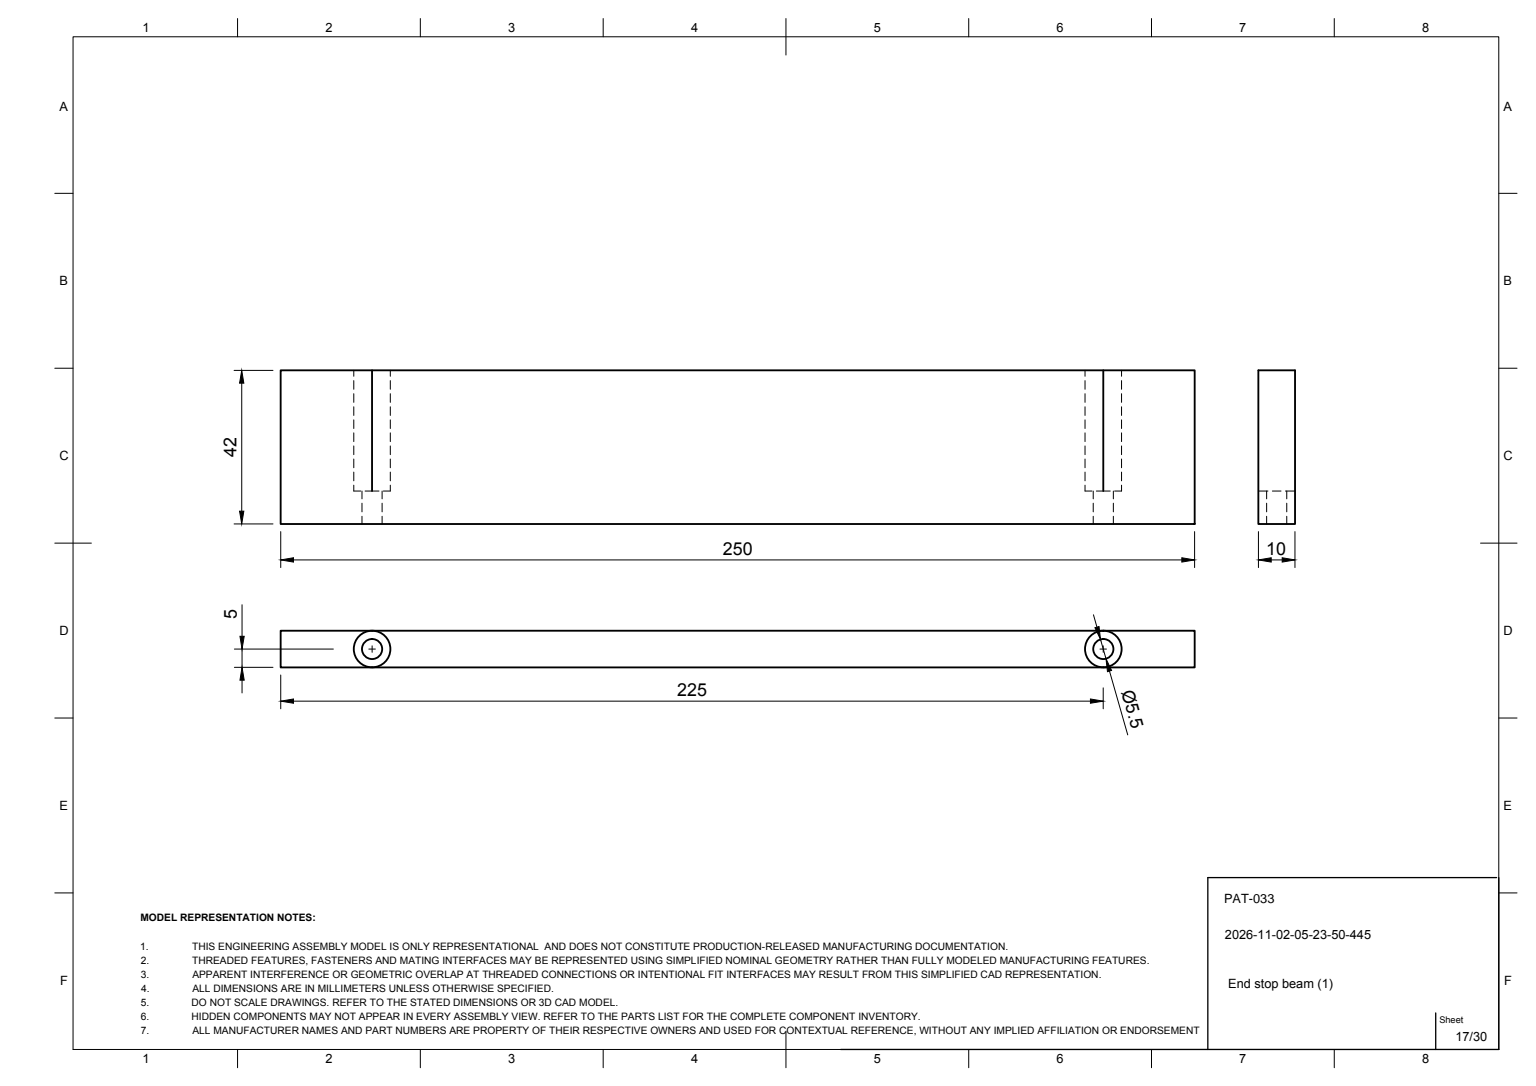
ISO-10303-21;
HEADER;
/* Generated by software containing ST-Developer
 * from STEP Tools, Inc. (www.steptools.com) 
 */

FILE_DESCRIPTION(
/* description */ ('Dual-rail gantry carriage'),
/* implementation_level */ '2;1');

FILE_NAME(
/* name */ 'End stop beam (1).step',
/* time_stamp */ '2026-10-27T10:49:15-07:00',
/* author */ (''),
/* organization */ (''),
/* preprocessor_version */ 'ST-DEVELOPER v20.2',
/* originating_system */ 'Autodesk Translation Framework v15.17.0.0',
/* authorisation */ '');

FILE_SCHEMA (('AUTOMOTIVE_DESIGN { 1 0 10303 214 3 1 1 }'));
ENDSEC;

DATA;
#10=MECHANICAL_DESIGN_GEOMETRIC_PRESENTATION_REPRESENTATION('',(#597),#12804);
#535=SHAPE_REPRESENTATION_RELATIONSHIP('SRR','None',#13013,#566);
#566=ADVANCED_BREP_SHAPE_REPRESENTATION('',(#628),#12783);
#597=STYLED_ITEM('',(#13233),#628);
#628=MANIFOLD_SOLID_BREP('Body1',#7375);
#686=FACE_BOUND('',#1586,.T.);
#687=FACE_BOUND('',#1590,.T.);
#688=FACE_BOUND('',#1601,.T.);
#689=FACE_BOUND('',#1602,.T.);
#840=PLANE('',#7916);
#841=PLANE('',#7924);
#842=PLANE('',#7926);
#843=PLANE('',#7927);
#844=PLANE('',#7928);
#845=PLANE('',#7933);
#846=PLANE('',#7934);
#847=PLANE('',#7935);
#848=PLANE('',#7936);
#849=PLANE('',#7937);
#1150=FACE_OUTER_BOUND('',#1583,.T.);
#1151=FACE_OUTER_BOUND('',#1584,.T.);
#1152=FACE_OUTER_BOUND('',#1585,.T.);
#1153=FACE_OUTER_BOUND('',#1587,.T.);
#1154=FACE_OUTER_BOUND('',#1588,.T.);
#1155=FACE_OUTER_BOUND('',#1589,.T.);
#1156=FACE_OUTER_BOUND('',#1591,.T.);
#1157=FACE_OUTER_BOUND('',#1592,.T.);
#1158=FACE_OUTER_BOUND('',#1593,.T.);
#1159=FACE_OUTER_BOUND('',#1594,.T.);
#1160=FACE_OUTER_BOUND('',#1595,.T.);
#1161=FACE_OUTER_BOUND('',#1596,.T.);
#1162=FACE_OUTER_BOUND('',#1597,.T.);
#1163=FACE_OUTER_BOUND('',#1598,.T.);
#1164=FACE_OUTER_BOUND('',#1599,.T.);
#1165=FACE_OUTER_BOUND('',#1600,.T.);
#1583=EDGE_LOOP('',(#5527,#5528,#5529,#5530));
#1584=EDGE_LOOP('',(#5531,#5532,#5533,#5534));
#1585=EDGE_LOOP('',(#5535,#5536));
#1586=EDGE_LOOP('',(#5537));
#1587=EDGE_LOOP('',(#5538,#5539,#5540,#5541));
#1588=EDGE_LOOP('',(#5542,#5543,#5544,#5545));
#1589=EDGE_LOOP('',(#5546,#5547));
#1590=EDGE_LOOP('',(#5548));
#1591=EDGE_LOOP('',(#5549,#5550,#5551,#5552));
#1592=EDGE_LOOP('',(#5553,#5554,#5555,#5556));
#1593=EDGE_LOOP('',(#5557,#5558,#5559,#5560));
#1594=EDGE_LOOP('',(#5561,#5562,#5563,#5564));
#1595=EDGE_LOOP('',(#5565,#5566,#5567,#5568));
#1596=EDGE_LOOP('',(#5569,#5570,#5571,#5572));
#1597=EDGE_LOOP('',(#5573,#5574,#5575,#5576,#5577,#5578,#5579,#5580,#5581,
#5582));
#1598=EDGE_LOOP('',(#5583,#5584,#5585,#5586));
#1599=EDGE_LOOP('',(#5587,#5588,#5589,#5590,#5591,#5592,#5593,#5594,#5595,
#5596));
#1600=EDGE_LOOP('',(#5597,#5598,#5599,#5600));
#1601=EDGE_LOOP('',(#5601));
#1602=EDGE_LOOP('',(#5602));
#2126=LINE('',#11186,#2835);
#2127=LINE('',#11190,#2836);
#2128=LINE('',#11193,#2837);
#2129=LINE('',#11195,#2838);
#2130=LINE('',#11203,#2839);
#2131=LINE('',#11207,#2840);
#2132=LINE('',#11210,#2841);
#2133=LINE('',#11212,#2842);
#2134=LINE('',#11219,#2843);
#2135=LINE('',#11221,#2844);
#2136=LINE('',#11222,#2845);
#2137=LINE('',#11224,#2846);
#2138=LINE('',#11225,#2847);
#2139=LINE('',#11228,#2848);
#2140=LINE('',#11230,#2849);
#2141=LINE('',#11231,#2850);
#2142=LINE('',#11235,#2851);
#2143=LINE('',#11239,#2852);
#2144=LINE('',#11243,#2853);
#2145=LINE('',#11244,#2854);
#2146=LINE('',#11245,#2855);
#2147=LINE('',#11248,#2856);
#2148=LINE('',#11249,#2857);
#2149=LINE('',#11252,#2858);
#2150=LINE('',#11253,#2859);
#2151=LINE('',#11255,#2860);
#2835=VECTOR('',#9005,1.);
#2836=VECTOR('',#9008,1.);
#2837=VECTOR('',#9013,1.);
#2838=VECTOR('',#9016,1.);
#2839=VECTOR('',#9025,1.);
#2840=VECTOR('',#9028,1.);
#2841=VECTOR('',#9033,1.);
#2842=VECTOR('',#9036,1.);
#2843=VECTOR('',#9045,1.);
#2844=VECTOR('',#9046,1.);
#2845=VECTOR('',#9047,1.);
#2846=VECTOR('',#9050,1.);
#2847=VECTOR('',#9051,1.);
#2848=VECTOR('',#9054,1.);
#2849=VECTOR('',#9055,1.);
#2850=VECTOR('',#9056,1.);
#2851=VECTOR('',#9061,0.274999999999999);
#2852=VECTOR('',#9066,0.274999999999999);
#2853=VECTOR('',#9069,1.);
#2854=VECTOR('',#9070,1.);
#2855=VECTOR('',#9071,1.);
#2856=VECTOR('',#9074,1.);
#2857=VECTOR('',#9075,1.);
#2858=VECTOR('',#9078,1.);
#2859=VECTOR('',#9079,1.);
#2860=VECTOR('',#9082,1.);
#3418=CIRCLE('',#7911,0.5);
#3419=CIRCLE('',#7912,0.5);
#3420=CIRCLE('',#7914,0.5);
#3421=CIRCLE('',#7915,0.5);
#3422=CIRCLE('',#7917,0.274999999999999);
#3423=CIRCLE('',#7919,0.5);
#3424=CIRCLE('',#7920,0.5);
#3425=CIRCLE('',#7922,0.5);
#3426=CIRCLE('',#7923,0.5);
#3427=CIRCLE('',#7925,0.274999999999999);
#3428=CIRCLE('',#7930,0.274999999999999);
#3429=CIRCLE('',#7932,0.274999999999999);
#3714=VERTEX_POINT('',#11184);
#3715=VERTEX_POINT('',#11185);
#3716=VERTEX_POINT('',#11187);
#3717=VERTEX_POINT('',#11189);
#3718=VERTEX_POINT('',#11198);
#3719=VERTEX_POINT('',#11201);
#3720=VERTEX_POINT('',#11202);
#3721=VERTEX_POINT('',#11204);
#3722=VERTEX_POINT('',#11206);
#3723=VERTEX_POINT('',#11215);
#3724=VERTEX_POINT('',#11218);
#3725=VERTEX_POINT('',#11220);
#3726=VERTEX_POINT('',#11227);
#3727=VERTEX_POINT('',#11229);
#3728=VERTEX_POINT('',#11233);
#3729=VERTEX_POINT('',#11237);
#3730=VERTEX_POINT('',#11241);
#3731=VERTEX_POINT('',#11242);
#3732=VERTEX_POINT('',#11247);
#3733=VERTEX_POINT('',#11251);
#4386=EDGE_CURVE('',#3714,#3715,#2126,.T.);
#4387=EDGE_CURVE('',#3716,#3715,#3418,.T.);
#4388=EDGE_CURVE('',#3717,#3716,#2127,.T.);
#4389=EDGE_CURVE('',#3714,#3717,#3419,.T.);
#4390=EDGE_CURVE('',#3714,#3715,#2128,.T.);
#4391=EDGE_CURVE('',#3717,#3714,#3420,.T.);
#4392=EDGE_CURVE('',#3717,#3716,#2129,.T.);
#4393=EDGE_CURVE('',#3715,#3716,#3421,.T.);
#4394=EDGE_CURVE('',#3718,#3718,#3422,.T.);
#4395=EDGE_CURVE('',#3719,#3720,#2130,.T.);
#4396=EDGE_CURVE('',#3721,#3720,#3423,.T.);
#4397=EDGE_CURVE('',#3722,#3721,#2131,.T.);
#4398=EDGE_CURVE('',#3719,#3722,#3424,.T.);
#4399=EDGE_CURVE('',#3719,#3720,#2132,.T.);
#4400=EDGE_CURVE('',#3722,#3719,#3425,.T.);
#4401=EDGE_CURVE('',#3722,#3721,#2133,.T.);
#4402=EDGE_CURVE('',#3720,#3721,#3426,.T.);
#4403=EDGE_CURVE('',#3723,#3723,#3427,.T.);
#4404=EDGE_CURVE('',#3720,#3724,#2134,.T.);
#4405=EDGE_CURVE('',#3724,#3725,#2135,.T.);
#4406=EDGE_CURVE('',#3725,#3721,#2136,.T.);
#4407=EDGE_CURVE('',#3715,#3720,#2137,.T.);
#4408=EDGE_CURVE('',#3721,#3716,#2138,.T.);
#4409=EDGE_CURVE('',#3716,#3726,#2139,.T.);
#4410=EDGE_CURVE('',#3726,#3727,#2140,.T.);
#4411=EDGE_CURVE('',#3727,#3715,#2141,.T.);
#4412=EDGE_CURVE('',#3728,#3728,#3428,.T.);
#4413=EDGE_CURVE('',#3728,#3718,#2142,.T.);
#4414=EDGE_CURVE('',#3729,#3729,#3429,.T.);
#4415=EDGE_CURVE('',#3729,#3723,#2143,.T.);
#4416=EDGE_CURVE('',#3730,#3731,#2144,.T.);
#4417=EDGE_CURVE('',#3731,#3725,#2145,.T.);
#4418=EDGE_CURVE('',#3730,#3724,#2146,.T.);
#4419=EDGE_CURVE('',#3732,#3730,#2147,.T.);
#4420=EDGE_CURVE('',#3732,#3727,#2148,.T.);
#4421=EDGE_CURVE('',#3733,#3732,#2149,.T.);
#4422=EDGE_CURVE('',#3733,#3726,#2150,.T.);
#4423=EDGE_CURVE('',#3731,#3733,#2151,.T.);
#5527=ORIENTED_EDGE('',*,*,#4386,.T.);
#5528=ORIENTED_EDGE('',*,*,#4387,.F.);
#5529=ORIENTED_EDGE('',*,*,#4388,.F.);
#5530=ORIENTED_EDGE('',*,*,#4389,.F.);
#5531=ORIENTED_EDGE('',*,*,#4390,.F.);
#5532=ORIENTED_EDGE('',*,*,#4391,.F.);
#5533=ORIENTED_EDGE('',*,*,#4392,.T.);
#5534=ORIENTED_EDGE('',*,*,#4393,.F.);
#5535=ORIENTED_EDGE('',*,*,#4391,.T.);
#5536=ORIENTED_EDGE('',*,*,#4389,.T.);
#5537=ORIENTED_EDGE('',*,*,#4394,.F.);
#5538=ORIENTED_EDGE('',*,*,#4395,.T.);
#5539=ORIENTED_EDGE('',*,*,#4396,.F.);
#5540=ORIENTED_EDGE('',*,*,#4397,.F.);
#5541=ORIENTED_EDGE('',*,*,#4398,.F.);
#5542=ORIENTED_EDGE('',*,*,#4399,.F.);
#5543=ORIENTED_EDGE('',*,*,#4400,.F.);
#5544=ORIENTED_EDGE('',*,*,#4401,.T.);
#5545=ORIENTED_EDGE('',*,*,#4402,.F.);
#5546=ORIENTED_EDGE('',*,*,#4400,.T.);
#5547=ORIENTED_EDGE('',*,*,#4398,.T.);
#5548=ORIENTED_EDGE('',*,*,#4403,.F.);
#5549=ORIENTED_EDGE('',*,*,#4396,.T.);
#5550=ORIENTED_EDGE('',*,*,#4404,.T.);
#5551=ORIENTED_EDGE('',*,*,#4405,.T.);
#5552=ORIENTED_EDGE('',*,*,#4406,.T.);
#5553=ORIENTED_EDGE('',*,*,#4387,.T.);
#5554=ORIENTED_EDGE('',*,*,#4407,.T.);
#5555=ORIENTED_EDGE('',*,*,#4402,.T.);
#5556=ORIENTED_EDGE('',*,*,#4408,.T.);
#5557=ORIENTED_EDGE('',*,*,#4393,.T.);
#5558=ORIENTED_EDGE('',*,*,#4409,.T.);
#5559=ORIENTED_EDGE('',*,*,#4410,.T.);
#5560=ORIENTED_EDGE('',*,*,#4411,.T.);
#5561=ORIENTED_EDGE('',*,*,#4412,.F.);
#5562=ORIENTED_EDGE('',*,*,#4413,.T.);
#5563=ORIENTED_EDGE('',*,*,#4394,.T.);
#5564=ORIENTED_EDGE('',*,*,#4413,.F.);
#5565=ORIENTED_EDGE('',*,*,#4414,.F.);
#5566=ORIENTED_EDGE('',*,*,#4415,.T.);
#5567=ORIENTED_EDGE('',*,*,#4403,.T.);
#5568=ORIENTED_EDGE('',*,*,#4415,.F.);
#5569=ORIENTED_EDGE('',*,*,#4416,.T.);
#5570=ORIENTED_EDGE('',*,*,#4417,.T.);
#5571=ORIENTED_EDGE('',*,*,#4405,.F.);
#5572=ORIENTED_EDGE('',*,*,#4418,.F.);
#5573=ORIENTED_EDGE('',*,*,#4419,.T.);
#5574=ORIENTED_EDGE('',*,*,#4418,.T.);
#5575=ORIENTED_EDGE('',*,*,#4404,.F.);
#5576=ORIENTED_EDGE('',*,*,#4395,.F.);
#5577=ORIENTED_EDGE('',*,*,#4399,.T.);
#5578=ORIENTED_EDGE('',*,*,#4407,.F.);
#5579=ORIENTED_EDGE('',*,*,#4386,.F.);
#5580=ORIENTED_EDGE('',*,*,#4390,.T.);
#5581=ORIENTED_EDGE('',*,*,#4411,.F.);
#5582=ORIENTED_EDGE('',*,*,#4420,.F.);
#5583=ORIENTED_EDGE('',*,*,#4421,.T.);
#5584=ORIENTED_EDGE('',*,*,#4420,.T.);
#5585=ORIENTED_EDGE('',*,*,#4410,.F.);
#5586=ORIENTED_EDGE('',*,*,#4422,.F.);
#5587=ORIENTED_EDGE('',*,*,#4423,.T.);
#5588=ORIENTED_EDGE('',*,*,#4422,.T.);
#5589=ORIENTED_EDGE('',*,*,#4409,.F.);
#5590=ORIENTED_EDGE('',*,*,#4392,.F.);
#5591=ORIENTED_EDGE('',*,*,#4388,.T.);
#5592=ORIENTED_EDGE('',*,*,#4408,.F.);
#5593=ORIENTED_EDGE('',*,*,#4401,.F.);
#5594=ORIENTED_EDGE('',*,*,#4397,.T.);
#5595=ORIENTED_EDGE('',*,*,#4406,.F.);
#5596=ORIENTED_EDGE('',*,*,#4417,.F.);
#5597=ORIENTED_EDGE('',*,*,#4423,.F.);
#5598=ORIENTED_EDGE('',*,*,#4416,.F.);
#5599=ORIENTED_EDGE('',*,*,#4419,.F.);
#5600=ORIENTED_EDGE('',*,*,#4421,.F.);
#5601=ORIENTED_EDGE('',*,*,#4412,.T.);
#5602=ORIENTED_EDGE('',*,*,#4414,.T.);
#6915=CYLINDRICAL_SURFACE('',#7910,0.5);
#6916=CYLINDRICAL_SURFACE('',#7913,0.5);
#6917=CYLINDRICAL_SURFACE('',#7918,0.5);
#6918=CYLINDRICAL_SURFACE('',#7921,0.5);
#6919=CYLINDRICAL_SURFACE('',#7929,0.274999999999999);
#6920=CYLINDRICAL_SURFACE('',#7931,0.274999999999999);
#7076=ADVANCED_FACE('',(#1150),#6915,.F.);
#7077=ADVANCED_FACE('',(#1151),#6916,.F.);
#7078=ADVANCED_FACE('',(#1152,#686),#840,.T.);
#7079=ADVANCED_FACE('',(#1153),#6917,.F.);
#7080=ADVANCED_FACE('',(#1154),#6918,.F.);
#7081=ADVANCED_FACE('',(#1155,#687),#841,.T.);
#7082=ADVANCED_FACE('',(#1156),#842,.T.);
#7083=ADVANCED_FACE('',(#1157),#843,.T.);
#7084=ADVANCED_FACE('',(#1158),#844,.T.);
#7085=ADVANCED_FACE('',(#1159),#6919,.F.);
#7086=ADVANCED_FACE('',(#1160),#6920,.F.);
#7087=ADVANCED_FACE('',(#1161),#845,.T.);
#7088=ADVANCED_FACE('',(#1162),#846,.T.);
#7089=ADVANCED_FACE('',(#1163),#847,.T.);
#7090=ADVANCED_FACE('',(#1164),#848,.T.);
#7091=ADVANCED_FACE('',(#1165,#688,#689),#849,.F.);
#7375=CLOSED_SHELL('',(#7076,#7077,#7078,#7079,#7080,#7081,#7082,#7083,
#7084,#7085,#7086,#7087,#7088,#7089,#7090,#7091));
#7909=AXIS2_PLACEMENT_3D('',#11182,#9001,#9002);
#7910=AXIS2_PLACEMENT_3D('',#11183,#9003,#9004);
#7911=AXIS2_PLACEMENT_3D('',#11188,#9006,#9007);
#7912=AXIS2_PLACEMENT_3D('',#11191,#9009,#9010);
#7913=AXIS2_PLACEMENT_3D('',#11192,#9011,#9012);
#7914=AXIS2_PLACEMENT_3D('',#11194,#9014,#9015);
#7915=AXIS2_PLACEMENT_3D('',#11196,#9017,#9018);
#7916=AXIS2_PLACEMENT_3D('',#11197,#9019,#9020);
#7917=AXIS2_PLACEMENT_3D('',#11199,#9021,#9022);
#7918=AXIS2_PLACEMENT_3D('',#11200,#9023,#9024);
#7919=AXIS2_PLACEMENT_3D('',#11205,#9026,#9027);
#7920=AXIS2_PLACEMENT_3D('',#11208,#9029,#9030);
#7921=AXIS2_PLACEMENT_3D('',#11209,#9031,#9032);
#7922=AXIS2_PLACEMENT_3D('',#11211,#9034,#9035);
#7923=AXIS2_PLACEMENT_3D('',#11213,#9037,#9038);
#7924=AXIS2_PLACEMENT_3D('',#11214,#9039,#9040);
#7925=AXIS2_PLACEMENT_3D('',#11216,#9041,#9042);
#7926=AXIS2_PLACEMENT_3D('',#11217,#9043,#9044);
#7927=AXIS2_PLACEMENT_3D('',#11223,#9048,#9049);
#7928=AXIS2_PLACEMENT_3D('',#11226,#9052,#9053);
#7929=AXIS2_PLACEMENT_3D('',#11232,#9057,#9058);
#7930=AXIS2_PLACEMENT_3D('',#11234,#9059,#9060);
#7931=AXIS2_PLACEMENT_3D('',#11236,#9062,#9063);
#7932=AXIS2_PLACEMENT_3D('',#11238,#9064,#9065);
#7933=AXIS2_PLACEMENT_3D('',#11240,#9067,#9068);
#7934=AXIS2_PLACEMENT_3D('',#11246,#9072,#9073);
#7935=AXIS2_PLACEMENT_3D('',#11250,#9076,#9077);
#7936=AXIS2_PLACEMENT_3D('',#11254,#9080,#9081);
#7937=AXIS2_PLACEMENT_3D('',#11256,#9083,#9084);
#9001=DIRECTION('axis',(0.,0.,1.));
#9002=DIRECTION('refdir',(1.,0.,0.));
#9003=DIRECTION('center_axis',(0.,0.,1.));
#9004=DIRECTION('ref_axis',(1.,0.,0.));
#9005=DIRECTION('',(0.,0.,1.));
#9006=DIRECTION('center_axis',(0.,0.,-1.));
#9007=DIRECTION('ref_axis',(1.,0.,0.));
#9008=DIRECTION('',(0.,0.,1.));
#9009=DIRECTION('center_axis',(0.,0.,1.));
#9010=DIRECTION('ref_axis',(1.,0.,0.));
#9011=DIRECTION('center_axis',(0.,0.,1.));
#9012=DIRECTION('ref_axis',(1.,0.,0.));
#9013=DIRECTION('',(0.,0.,1.));
#9014=DIRECTION('center_axis',(0.,0.,1.));
#9015=DIRECTION('ref_axis',(1.,0.,0.));
#9016=DIRECTION('',(0.,0.,1.));
#9017=DIRECTION('center_axis',(0.,0.,-1.));
#9018=DIRECTION('ref_axis',(1.,0.,0.));
#9019=DIRECTION('center_axis',(0.,0.,1.));
#9020=DIRECTION('ref_axis',(1.,0.,0.));
#9021=DIRECTION('center_axis',(0.,0.,1.));
#9022=DIRECTION('ref_axis',(1.,0.,0.));
#9023=DIRECTION('center_axis',(0.,0.,1.));
#9024=DIRECTION('ref_axis',(1.,0.,0.));
#9025=DIRECTION('',(0.,0.,1.));
#9026=DIRECTION('center_axis',(0.,0.,-1.));
#9027=DIRECTION('ref_axis',(1.,0.,0.));
#9028=DIRECTION('',(0.,0.,1.));
#9029=DIRECTION('center_axis',(0.,0.,1.));
#9030=DIRECTION('ref_axis',(1.,0.,0.));
#9031=DIRECTION('center_axis',(0.,0.,1.));
#9032=DIRECTION('ref_axis',(1.,0.,0.));
#9033=DIRECTION('',(0.,0.,1.));
#9034=DIRECTION('center_axis',(0.,0.,1.));
#9035=DIRECTION('ref_axis',(1.,0.,0.));
#9036=DIRECTION('',(0.,0.,1.));
#9037=DIRECTION('center_axis',(0.,0.,-1.));
#9038=DIRECTION('ref_axis',(1.,0.,0.));
#9039=DIRECTION('center_axis',(0.,0.,1.));
#9040=DIRECTION('ref_axis',(1.,0.,0.));
#9041=DIRECTION('center_axis',(0.,0.,1.));
#9042=DIRECTION('ref_axis',(1.,0.,0.));
#9043=DIRECTION('center_axis',(0.,0.,1.));
#9044=DIRECTION('ref_axis',(1.,0.,0.));
#9045=DIRECTION('',(0.,1.,0.));
#9046=DIRECTION('',(-1.,0.,0.));
#9047=DIRECTION('',(0.,-1.,0.));
#9048=DIRECTION('center_axis',(0.,0.,1.));
#9049=DIRECTION('ref_axis',(1.,0.,0.));
#9050=DIRECTION('',(0.,1.,0.));
#9051=DIRECTION('',(0.,-1.,0.));
#9052=DIRECTION('center_axis',(0.,0.,1.));
#9053=DIRECTION('ref_axis',(1.,0.,0.));
#9054=DIRECTION('',(0.,-1.,0.));
#9055=DIRECTION('',(1.,0.,0.));
#9056=DIRECTION('',(0.,1.,0.));
#9057=DIRECTION('center_axis',(0.,0.,1.));
#9058=DIRECTION('ref_axis',(1.,0.,0.));
#9059=DIRECTION('center_axis',(0.,0.,1.));
#9060=DIRECTION('ref_axis',(1.,0.,0.));
#9061=DIRECTION('',(0.,0.,1.));
#9062=DIRECTION('center_axis',(0.,0.,1.));
#9063=DIRECTION('ref_axis',(1.,0.,0.));
#9064=DIRECTION('center_axis',(0.,0.,1.));
#9065=DIRECTION('ref_axis',(1.,0.,0.));
#9066=DIRECTION('',(0.,0.,1.));
#9067=DIRECTION('center_axis',(0.,1.,0.));
#9068=DIRECTION('ref_axis',(-1.,0.,0.));
#9069=DIRECTION('',(-1.,0.,0.));
#9070=DIRECTION('',(0.,0.,1.));
#9071=DIRECTION('',(0.,0.,1.));
#9072=DIRECTION('center_axis',(1.,0.,0.));
#9073=DIRECTION('ref_axis',(0.,1.,0.));
#9074=DIRECTION('',(0.,1.,0.));
#9075=DIRECTION('',(0.,0.,1.));
#9076=DIRECTION('center_axis',(0.,-1.,0.));
#9077=DIRECTION('ref_axis',(1.,0.,0.));
#9078=DIRECTION('',(1.,0.,0.));
#9079=DIRECTION('',(0.,0.,1.));
#9080=DIRECTION('center_axis',(-1.,0.,0.));
#9081=DIRECTION('ref_axis',(0.,-1.,0.));
#9082=DIRECTION('',(0.,-1.,0.));
#9083=DIRECTION('center_axis',(0.,0.,1.));
#9084=DIRECTION('ref_axis',(1.,0.,0.));
#11182=CARTESIAN_POINT('',(0.,0.,0.));
#11183=CARTESIAN_POINT('Origin',(32.5,-10.,2.9));
#11184=CARTESIAN_POINT('',(33.,-10.,2.9));
#11185=CARTESIAN_POINT('',(33.,-10.,6.2));
#11186=CARTESIAN_POINT('',(33.,-10.,2.9));
#11187=CARTESIAN_POINT('',(32.,-10.,6.2));
#11188=CARTESIAN_POINT('Origin',(32.5,-10.,6.2));
#11189=CARTESIAN_POINT('',(32.,-10.,2.9));
#11190=CARTESIAN_POINT('',(32.,-10.,2.9));
#11191=CARTESIAN_POINT('Origin',(32.5,-10.,2.9));
#11192=CARTESIAN_POINT('Origin',(32.5,-10.,2.9));
#11193=CARTESIAN_POINT('',(33.,-10.,2.9));
#11194=CARTESIAN_POINT('Origin',(32.5,-10.,2.9));
#11195=CARTESIAN_POINT('',(32.,-10.,2.9));
#11196=CARTESIAN_POINT('Origin',(32.5,-10.,6.2));
#11197=CARTESIAN_POINT('Origin',(32.5,-10.,2.9));
#11198=CARTESIAN_POINT('',(32.225,-10.,2.9));
#11199=CARTESIAN_POINT('Origin',(32.5,-10.,2.9));
#11200=CARTESIAN_POINT('Origin',(32.5,10.,2.9));
#11201=CARTESIAN_POINT('',(33.,10.,2.9));
#11202=CARTESIAN_POINT('',(33.,10.,6.2));
#11203=CARTESIAN_POINT('',(33.,10.,2.9));
#11204=CARTESIAN_POINT('',(32.,10.,6.2));
#11205=CARTESIAN_POINT('Origin',(32.5,10.,6.2));
#11206=CARTESIAN_POINT('',(32.,10.,2.9));
#11207=CARTESIAN_POINT('',(32.,10.,2.9));
#11208=CARTESIAN_POINT('Origin',(32.5,10.,2.9));
#11209=CARTESIAN_POINT('Origin',(32.5,10.,2.9));
#11210=CARTESIAN_POINT('',(33.,10.,2.9));
#11211=CARTESIAN_POINT('Origin',(32.5,10.,2.9));
#11212=CARTESIAN_POINT('',(32.,10.,2.9));
#11213=CARTESIAN_POINT('Origin',(32.5,10.,6.2));
#11214=CARTESIAN_POINT('Origin',(32.5,10.,2.9));
#11215=CARTESIAN_POINT('',(32.225,10.,2.9));
#11216=CARTESIAN_POINT('Origin',(32.5,10.,2.9));
#11217=CARTESIAN_POINT('Origin',(32.5,0.,6.2));
#11218=CARTESIAN_POINT('',(33.,12.5,6.2));
#11219=CARTESIAN_POINT('',(33.,-12.5,6.2));
#11220=CARTESIAN_POINT('',(32.,12.5,6.2));
#11221=CARTESIAN_POINT('',(33.,12.5,6.2));
#11222=CARTESIAN_POINT('',(32.,12.5,6.2));
#11223=CARTESIAN_POINT('Origin',(32.5,0.,6.2));
#11224=CARTESIAN_POINT('',(33.,-12.5,6.2));
#11225=CARTESIAN_POINT('',(32.,12.5,6.2));
#11226=CARTESIAN_POINT('Origin',(32.5,0.,6.2));
#11227=CARTESIAN_POINT('',(32.,-12.5,6.2));
#11228=CARTESIAN_POINT('',(32.,12.5,6.2));
#11229=CARTESIAN_POINT('',(33.,-12.5,6.2));
#11230=CARTESIAN_POINT('',(32.,-12.5,6.2));
#11231=CARTESIAN_POINT('',(33.,-12.5,6.2));
#11232=CARTESIAN_POINT('Origin',(32.5,-10.,1.9));
#11233=CARTESIAN_POINT('',(32.225,-10.,2.));
#11234=CARTESIAN_POINT('Origin',(32.5,-10.,2.));
#11235=CARTESIAN_POINT('',(32.225,-10.,1.9));
#11236=CARTESIAN_POINT('Origin',(32.5,10.,1.9));
#11237=CARTESIAN_POINT('',(32.225,10.,2.));
#11238=CARTESIAN_POINT('Origin',(32.5,10.,2.));
#11239=CARTESIAN_POINT('',(32.225,10.,1.9));
#11240=CARTESIAN_POINT('Origin',(33.,12.5,2.));
#11241=CARTESIAN_POINT('',(33.,12.5,2.));
#11242=CARTESIAN_POINT('',(32.,12.5,2.));
#11243=CARTESIAN_POINT('',(33.,12.5,2.));
#11244=CARTESIAN_POINT('',(32.,12.5,2.));
#11245=CARTESIAN_POINT('',(33.,12.5,2.));
#11246=CARTESIAN_POINT('Origin',(33.,-12.5,2.));
#11247=CARTESIAN_POINT('',(33.,-12.5,2.));
#11248=CARTESIAN_POINT('',(33.,-12.5,2.));
#11249=CARTESIAN_POINT('',(33.,-12.5,2.));
#11250=CARTESIAN_POINT('Origin',(32.,-12.5,2.));
#11251=CARTESIAN_POINT('',(32.,-12.5,2.));
#11252=CARTESIAN_POINT('',(32.,-12.5,2.));
#11253=CARTESIAN_POINT('',(32.,-12.5,2.));
#11254=CARTESIAN_POINT('Origin',(32.,12.5,2.));
#11255=CARTESIAN_POINT('',(32.,12.5,2.));
#11256=CARTESIAN_POINT('Origin',(32.5,0.,2.));
#12747=UNCERTAINTY_MEASURE_WITH_UNIT(LENGTH_MEASURE(0.001),#12805,
'DISTANCE_ACCURACY_VALUE',
'Maximum model space distance between geometric entities at asserted c
onnectivities');
#12768=UNCERTAINTY_MEASURE_WITH_UNIT(LENGTH_MEASURE(0.001),#12805,
'DISTANCE_ACCURACY_VALUE',
'Maximum model space distance between geometric entities at asserted c
onnectivities');
#12783=(
GEOMETRIC_REPRESENTATION_CONTEXT(3)
GLOBAL_UNCERTAINTY_ASSIGNED_CONTEXT((#12747))
GLOBAL_UNIT_ASSIGNED_CONTEXT((#12805,#12807,#12808))
REPRESENTATION_CONTEXT('','3D')
);
#12804=(
GEOMETRIC_REPRESENTATION_CONTEXT(3)
GLOBAL_UNCERTAINTY_ASSIGNED_CONTEXT((#12768))
GLOBAL_UNIT_ASSIGNED_CONTEXT((#12805,#12807,#12808))
REPRESENTATION_CONTEXT('','3D')
);
#12805=(
LENGTH_UNIT()
NAMED_UNIT(*)
SI_UNIT(.CENTI.,.METRE.)
);
#12807=(
NAMED_UNIT(*)
PLANE_ANGLE_UNIT()
SI_UNIT($,.RADIAN.)
);
#12808=(
NAMED_UNIT(*)
SI_UNIT($,.STERADIAN.)
SOLID_ANGLE_UNIT()
);
#12823=SHAPE_DEFINITION_REPRESENTATION(#12858,#13013);
#12858=PRODUCT_DEFINITION_SHAPE('',$,#13049);
#13013=SHAPE_REPRESENTATION('',(#7909),#12783);
#13034=PRODUCT_DEFINITION_CONTEXT('part definition',#13141,'design');
#13049=PRODUCT_DEFINITION('End stop beam (1)','End stop beam (1)',#13084,
#13034);
#13084=PRODUCT_DEFINITION_FORMATION('',$,#13157);
#13141=APPLICATION_CONTEXT(
'Core Data for Automotive Mechanical Design Process');
#13142=PRODUCT_CONTEXT('part definition',#13141,'mechanical');
#13157=PRODUCT('End stop beam (1)','End stop beam (1)','End stop beam (1)',(#13142));
#13227=COLOUR_RGB('Light Blue',0.38,0.62,0.78);
#13228=FILL_AREA_STYLE_COLOUR('',#13227);
#13229=FILL_AREA_STYLE('',(#13228));
#13230=SURFACE_STYLE_FILL_AREA(#13229);
#13231=SURFACE_SIDE_STYLE('',(#13230));
#13232=SURFACE_STYLE_USAGE(.BOTH.,#13231);
#13233=PRESENTATION_STYLE_ASSIGNMENT((#13232));
ENDSEC;
END-ISO-10303-21;
